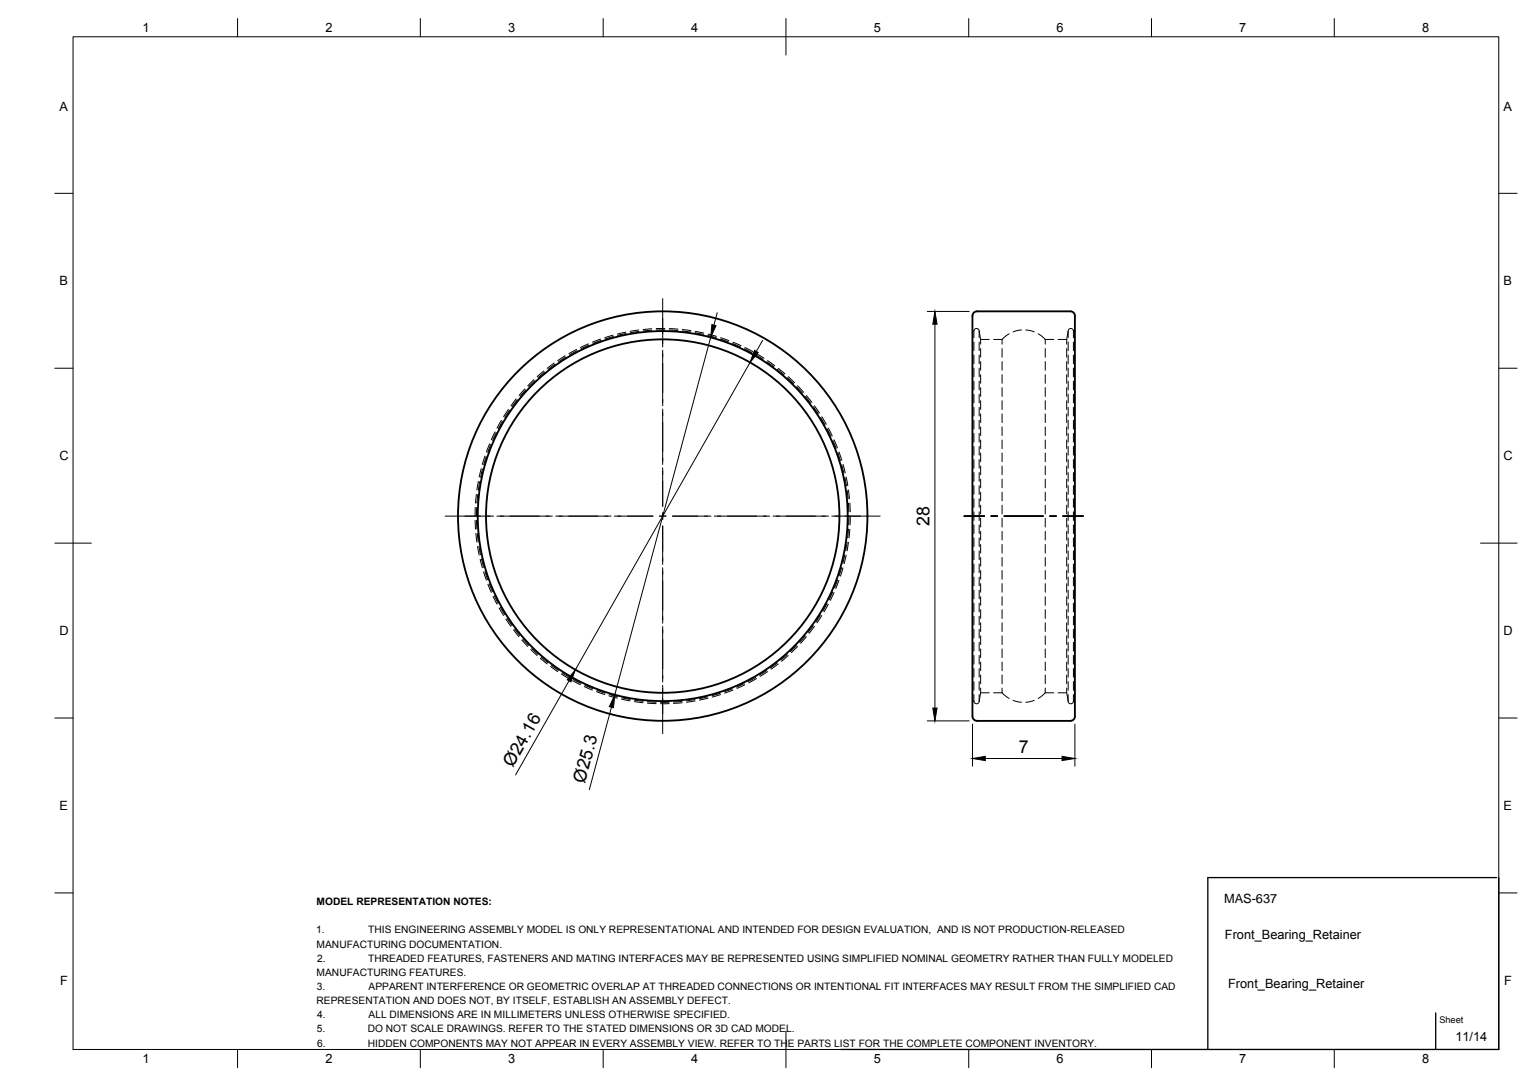
ISO-10303-21;
HEADER;
FILE_DESCRIPTION((''),'2;1');
FILE_NAME('Front_Bearing_Retainer.step','2026-10-09T10:11:57-07:00',(''),(''),'','','');
FILE_SCHEMA (('AUTOMOTIVE_DESIGN { 1 0 10303 214 3 1 1 }'));
ENDSEC;
DATA;
#10=MECHANICAL_DESIGN_GEOMETRIC_PRESENTATION_REPRESENTATION('',(#143),#13510);
#104=SHAPE_REPRESENTATION_RELATIONSHIP('SRR','None',#13574,#119) ;
#119=ADVANCED_BREP_SHAPE_REPRESENTATION('',(#175),#13506) ;
#143=STYLED_ITEM('',(#13650),#175) ;
#175=MANIFOLD_SOLID_BREP('Body1',#7392) ;
#254=FACE_BOUND('',#1570,.T.) ;
#255=FACE_BOUND('',#1572,.T.) ;
#462=PLANE('',#8395) ;
#463=PLANE('',#8396) ;
#516=TOROIDAL_SURFACE('',#8373,12.65,0.18) ;
#517=TOROIDAL_SURFACE('',#8378,13.7,0.3) ;
#518=TOROIDAL_SURFACE('',#8384,13.7,0.3) ;
#519=TOROIDAL_SURFACE('',#8390,12.65,0.18) ;
#520=TOROIDAL_SURFACE('',#8401,10.75,1.985) ;
#651=CYLINDRICAL_SURFACE('',#8376,12.65) ;
#652=CYLINDRICAL_SURFACE('',#8382,14.) ;
#653=CYLINDRICAL_SURFACE('',#8387,12.65) ;
#654=CYLINDRICAL_SURFACE('',#8397,12.08) ;
#655=CYLINDRICAL_SURFACE('',#8399,12.08) ;
#1045=FACE_OUTER_BOUND('',#1560,.T.) ;
#1046=FACE_OUTER_BOUND('',#1561,.T.) ;
#1047=FACE_OUTER_BOUND('',#1562,.T.) ;
#1048=FACE_OUTER_BOUND('',#1563,.T.) ;
#1049=FACE_OUTER_BOUND('',#1564,.T.) ;
#1050=FACE_OUTER_BOUND('',#1565,.T.) ;
#1051=FACE_OUTER_BOUND('',#1566,.T.) ;
#1052=FACE_OUTER_BOUND('',#1567,.T.) ;
#1053=FACE_OUTER_BOUND('',#1568,.T.) ;
#1054=FACE_OUTER_BOUND('',#1569,.T.) ;
#1055=FACE_OUTER_BOUND('',#1571,.T.) ;
#1056=FACE_OUTER_BOUND('',#1573,.T.) ;
#1057=FACE_OUTER_BOUND('',#1574,.T.) ;
#1058=FACE_OUTER_BOUND('',#1575,.T.) ;
#1560=EDGE_LOOP('',(#6604,#6605,#6606,#6607)) ;
#1561=EDGE_LOOP('',(#6608,#6609,#6610,#6611)) ;
#1562=EDGE_LOOP('',(#6612,#6613,#6614,#6615)) ;
#1563=EDGE_LOOP('',(#6616,#6617,#6618,#6619)) ;
#1564=EDGE_LOOP('',(#6620,#6621,#6622,#6623)) ;
#1565=EDGE_LOOP('',(#6624,#6625,#6626,#6627)) ;
#1566=EDGE_LOOP('',(#6628,#6629,#6630,#6631)) ;
#1567=EDGE_LOOP('',(#6632,#6633,#6634,#6635)) ;
#1568=EDGE_LOOP('',(#6636,#6637,#6638,#6639)) ;
#1569=EDGE_LOOP('',(#6640)) ;
#1570=EDGE_LOOP('',(#6641)) ;
#1571=EDGE_LOOP('',(#6642)) ;
#1572=EDGE_LOOP('',(#6643)) ;
#1573=EDGE_LOOP('',(#6644,#6645,#6646,#6647)) ;
#1574=EDGE_LOOP('',(#6648,#6649,#6650,#6651)) ;
#1575=EDGE_LOOP('',(#6652,#6653,#6654,#6655)) ;
#2112=LINE('',#13167,#2606) ;
#2113=LINE('',#13176,#2607) ;
#2114=LINE('',#13186,#2608) ;
#2115=LINE('',#13195,#2609) ;
#2116=LINE('',#13204,#2610) ;
#2117=LINE('',#13210,#2611) ;
#2118=LINE('',#13213,#2612) ;
#2606=VECTOR('',#10634,12.08) ;
#2607=VECTOR('',#10647,12.65) ;
#2608=VECTOR('',#10660,14.) ;
#2609=VECTOR('',#10671,12.65) ;
#2610=VECTOR('',#10684,12.08) ;
#2611=VECTOR('',#10693,12.08) ;
#2612=VECTOR('',#10696,12.08) ;
#3041=CIRCLE('',#8371,12.08) ;
#3042=CIRCLE('',#8372,12.65) ;
#3043=CIRCLE('',#8374,12.65) ;
#3044=CIRCLE('',#8375,0.18) ;
#3045=CIRCLE('',#8377,12.65) ;
#3046=CIRCLE('',#8379,14.) ;
#3047=CIRCLE('',#8380,0.3) ;
#3048=CIRCLE('',#8381,13.7) ;
#3049=CIRCLE('',#8383,14.) ;
#3050=CIRCLE('',#8385,13.7) ;
#3051=CIRCLE('',#8386,0.3) ;
#3052=CIRCLE('',#8388,12.65) ;
#3053=CIRCLE('',#8389,12.65) ;
#3054=CIRCLE('',#8391,12.65) ;
#3055=CIRCLE('',#8392,0.18) ;
#3056=CIRCLE('',#8394,12.08) ;
#3057=CIRCLE('',#8398,12.08) ;
#3058=CIRCLE('',#8400,12.08) ;
#3059=CIRCLE('',#8402,1.985) ;
#3712=VERTEX_POINT('',#13164) ;
#3713=VERTEX_POINT('',#13166) ;
#3714=VERTEX_POINT('',#13170) ;
#3715=VERTEX_POINT('',#13174) ;
#3716=VERTEX_POINT('',#13178) ;
#3717=VERTEX_POINT('',#13180) ;
#3718=VERTEX_POINT('',#13184) ;
#3719=VERTEX_POINT('',#13188) ;
#3720=VERTEX_POINT('',#13192) ;
#3721=VERTEX_POINT('',#13194) ;
#3722=VERTEX_POINT('',#13198) ;
#3723=VERTEX_POINT('',#13202) ;
#3724=VERTEX_POINT('',#13208) ;
#3725=VERTEX_POINT('',#13212) ;
#4689=EDGE_CURVE('',#3712,#3712,#3041,.F.) ;
#4690=EDGE_CURVE('',#3712,#3713,#2112,.T.) ;
#4691=EDGE_CURVE('',#3713,#3713,#3042,.F.) ;
#4692=EDGE_CURVE('',#3714,#3714,#3043,.T.) ;
#4693=EDGE_CURVE('',#3714,#3713,#3044,.T.) ;
#4694=EDGE_CURVE('',#3715,#3715,#3045,.T.) ;
#4695=EDGE_CURVE('',#3715,#3714,#2113,.T.) ;
#4696=EDGE_CURVE('',#3716,#3716,#3046,.T.) ;
#4697=EDGE_CURVE('',#3716,#3717,#3047,.T.) ;
#4698=EDGE_CURVE('',#3717,#3717,#3048,.T.) ;
#4699=EDGE_CURVE('',#3718,#3718,#3049,.T.) ;
#4700=EDGE_CURVE('',#3718,#3716,#2114,.T.) ;
#4701=EDGE_CURVE('',#3719,#3719,#3050,.T.) ;
#4702=EDGE_CURVE('',#3719,#3718,#3051,.T.) ;
#4703=EDGE_CURVE('',#3720,#3720,#3052,.T.) ;
#4704=EDGE_CURVE('',#3720,#3721,#2115,.T.) ;
#4705=EDGE_CURVE('',#3721,#3721,#3053,.T.) ;
#4706=EDGE_CURVE('',#3722,#3722,#3054,.T.) ;
#4707=EDGE_CURVE('',#3722,#3720,#3055,.T.) ;
#4708=EDGE_CURVE('',#3723,#3723,#3056,.T.) ;
#4709=EDGE_CURVE('',#3723,#3722,#2116,.T.) ;
#4710=EDGE_CURVE('',#3724,#3724,#3057,.T.) ;
#4711=EDGE_CURVE('',#3724,#3723,#2117,.T.) ;
#4712=EDGE_CURVE('',#3712,#3725,#2118,.T.) ;
#4713=EDGE_CURVE('',#3725,#3725,#3058,.T.) ;
#4714=EDGE_CURVE('',#3725,#3724,#3059,.T.) ;
#6604=ORIENTED_EDGE('',*,*,#4689,.T.) ;
#6605=ORIENTED_EDGE('',*,*,#4690,.T.) ;
#6606=ORIENTED_EDGE('',*,*,#4691,.F.) ;
#6607=ORIENTED_EDGE('',*,*,#4690,.F.) ;
#6608=ORIENTED_EDGE('',*,*,#4692,.F.) ;
#6609=ORIENTED_EDGE('',*,*,#4693,.T.) ;
#6610=ORIENTED_EDGE('',*,*,#4691,.T.) ;
#6611=ORIENTED_EDGE('',*,*,#4693,.F.) ;
#6612=ORIENTED_EDGE('',*,*,#4694,.F.) ;
#6613=ORIENTED_EDGE('',*,*,#4695,.T.) ;
#6614=ORIENTED_EDGE('',*,*,#4692,.T.) ;
#6615=ORIENTED_EDGE('',*,*,#4695,.F.) ;
#6616=ORIENTED_EDGE('',*,*,#4696,.F.) ;
#6617=ORIENTED_EDGE('',*,*,#4697,.T.) ;
#6618=ORIENTED_EDGE('',*,*,#4698,.T.) ;
#6619=ORIENTED_EDGE('',*,*,#4697,.F.) ;
#6620=ORIENTED_EDGE('',*,*,#4699,.F.) ;
#6621=ORIENTED_EDGE('',*,*,#4700,.T.) ;
#6622=ORIENTED_EDGE('',*,*,#4696,.T.) ;
#6623=ORIENTED_EDGE('',*,*,#4700,.F.) ;
#6624=ORIENTED_EDGE('',*,*,#4701,.F.) ;
#6625=ORIENTED_EDGE('',*,*,#4702,.T.) ;
#6626=ORIENTED_EDGE('',*,*,#4699,.T.) ;
#6627=ORIENTED_EDGE('',*,*,#4702,.F.) ;
#6628=ORIENTED_EDGE('',*,*,#4703,.F.) ;
#6629=ORIENTED_EDGE('',*,*,#4704,.T.) ;
#6630=ORIENTED_EDGE('',*,*,#4705,.T.) ;
#6631=ORIENTED_EDGE('',*,*,#4704,.F.) ;
#6632=ORIENTED_EDGE('',*,*,#4706,.F.) ;
#6633=ORIENTED_EDGE('',*,*,#4707,.T.) ;
#6634=ORIENTED_EDGE('',*,*,#4703,.T.) ;
#6635=ORIENTED_EDGE('',*,*,#4707,.F.) ;
#6636=ORIENTED_EDGE('',*,*,#4708,.F.) ;
#6637=ORIENTED_EDGE('',*,*,#4709,.T.) ;
#6638=ORIENTED_EDGE('',*,*,#4706,.T.) ;
#6639=ORIENTED_EDGE('',*,*,#4709,.F.) ;
#6640=ORIENTED_EDGE('',*,*,#4698,.F.) ;
#6641=ORIENTED_EDGE('',*,*,#4694,.T.) ;
#6642=ORIENTED_EDGE('',*,*,#4701,.T.) ;
#6643=ORIENTED_EDGE('',*,*,#4705,.F.) ;
#6644=ORIENTED_EDGE('',*,*,#4710,.F.) ;
#6645=ORIENTED_EDGE('',*,*,#4711,.T.) ;
#6646=ORIENTED_EDGE('',*,*,#4708,.T.) ;
#6647=ORIENTED_EDGE('',*,*,#4711,.F.) ;
#6648=ORIENTED_EDGE('',*,*,#4689,.F.) ;
#6649=ORIENTED_EDGE('',*,*,#4712,.T.) ;
#6650=ORIENTED_EDGE('',*,*,#4713,.T.) ;
#6651=ORIENTED_EDGE('',*,*,#4712,.F.) ;
#6652=ORIENTED_EDGE('',*,*,#4713,.F.) ;
#6653=ORIENTED_EDGE('',*,*,#4714,.T.) ;
#6654=ORIENTED_EDGE('',*,*,#4710,.T.) ;
#6655=ORIENTED_EDGE('',*,*,#4714,.F.) ;
#6904=CONICAL_SURFACE('',#8370,12.08,1.3962634016) ;
#6905=CONICAL_SURFACE('',#8393,12.08,1.3962634016) ;
#7295=ADVANCED_FACE('',(#1045),#6904,.F.) ;
#7296=ADVANCED_FACE('',(#1046),#516,.F.) ;
#7297=ADVANCED_FACE('',(#1047),#651,.F.) ;
#7298=ADVANCED_FACE('',(#1048),#517,.T.) ;
#7299=ADVANCED_FACE('',(#1049),#652,.T.) ;
#7300=ADVANCED_FACE('',(#1050),#518,.T.) ;
#7301=ADVANCED_FACE('',(#1051),#653,.F.) ;
#7302=ADVANCED_FACE('',(#1052),#519,.F.) ;
#7303=ADVANCED_FACE('',(#1053),#6905,.F.) ;
#7304=ADVANCED_FACE('',(#1054,#254),#462,.F.) ;
#7305=ADVANCED_FACE('',(#1055,#255),#463,.T.) ;
#7306=ADVANCED_FACE('',(#1056),#654,.F.) ;
#7307=ADVANCED_FACE('',(#1057),#655,.F.) ;
#7308=ADVANCED_FACE('',(#1058),#520,.F.) ;
#7392=CLOSED_SHELL('',(#7295,#7296,#7297,#7298,#7299,#7300,#7301,#7302,
#7303,#7304,#7305,#7306,#7307,#7308)) ;
#8369=AXIS2_PLACEMENT_3D('',#13162,#10628,#10629) ;
#8370=AXIS2_PLACEMENT_3D('',#13163,#10630,#10631) ;
#8371=AXIS2_PLACEMENT_3D('',#13165,#10632,#10633) ;
#8372=AXIS2_PLACEMENT_3D('',#13168,#10635,#10636) ;
#8373=AXIS2_PLACEMENT_3D('',#13169,#10637,#10638) ;
#8374=AXIS2_PLACEMENT_3D('',#13171,#10639,#10640) ;
#8375=AXIS2_PLACEMENT_3D('',#13172,#10641,#10642) ;
#8376=AXIS2_PLACEMENT_3D('',#13173,#10643,#10644) ;
#8377=AXIS2_PLACEMENT_3D('',#13175,#10645,#10646) ;
#8378=AXIS2_PLACEMENT_3D('',#13177,#10648,#10649) ;
#8379=AXIS2_PLACEMENT_3D('',#13179,#10650,#10651) ;
#8380=AXIS2_PLACEMENT_3D('',#13181,#10652,#10653) ;
#8381=AXIS2_PLACEMENT_3D('',#13182,#10654,#10655) ;
#8382=AXIS2_PLACEMENT_3D('',#13183,#10656,#10657) ;
#8383=AXIS2_PLACEMENT_3D('',#13185,#10658,#10659) ;
#8384=AXIS2_PLACEMENT_3D('',#13187,#10661,#10662) ;
#8385=AXIS2_PLACEMENT_3D('',#13189,#10663,#10664) ;
#8386=AXIS2_PLACEMENT_3D('',#13190,#10665,#10666) ;
#8387=AXIS2_PLACEMENT_3D('',#13191,#10667,#10668) ;
#8388=AXIS2_PLACEMENT_3D('',#13193,#10669,#10670) ;
#8389=AXIS2_PLACEMENT_3D('',#13196,#10672,#10673) ;
#8390=AXIS2_PLACEMENT_3D('',#13197,#10674,#10675) ;
#8391=AXIS2_PLACEMENT_3D('',#13199,#10676,#10677) ;
#8392=AXIS2_PLACEMENT_3D('',#13200,#10678,#10679) ;
#8393=AXIS2_PLACEMENT_3D('',#13201,#10680,#10681) ;
#8394=AXIS2_PLACEMENT_3D('',#13203,#10682,#10683) ;
#8395=AXIS2_PLACEMENT_3D('',#13205,#10685,#10686) ;
#8396=AXIS2_PLACEMENT_3D('',#13206,#10687,#10688) ;
#8397=AXIS2_PLACEMENT_3D('',#13207,#10689,#10690) ;
#8398=AXIS2_PLACEMENT_3D('',#13209,#10691,#10692) ;
#8399=AXIS2_PLACEMENT_3D('',#13211,#10694,#10695) ;
#8400=AXIS2_PLACEMENT_3D('',#13214,#10697,#10698) ;
#8401=AXIS2_PLACEMENT_3D('',#13215,#10699,#10700) ;
#8402=AXIS2_PLACEMENT_3D('',#13216,#10701,#10702) ;
#10628=DIRECTION('axis',(0.,0.,1.)) ;
#10629=DIRECTION('refdir',(1.,0.,0.)) ;
#10630=DIRECTION('center_axis',(0.,0.,1.)) ;
#10631=DIRECTION('ref_axis',(0.877582561890372,-0.479425538604204,0.)) ;
#10632=DIRECTION('center_axis',(0.,0.,1.)) ;
#10633=DIRECTION('ref_axis',(-1.,0.,0.)) ;
#10634=DIRECTION('',(-0.864250110858646,0.472141987409851,0.173648177662463)) ;
#10635=DIRECTION('center_axis',(0.,0.,1.)) ;
#10636=DIRECTION('ref_axis',(-1.,0.,0.)) ;
#10637=DIRECTION('center_axis',(0.,0.,-1.)) ;
#10638=DIRECTION('ref_axis',(0.877582561890372,-0.479425538604204,0.)) ;
#10639=DIRECTION('center_axis',(0.,0.,-1.)) ;
#10640=DIRECTION('ref_axis',(1.,0.,0.)) ;
#10641=DIRECTION('center_axis',(-0.479425538604204,-0.877582561890372,0.)) ;
#10642=DIRECTION('ref_axis',(-0.877582561890372,0.479425538604204,0.)) ;
#10643=DIRECTION('center_axis',(0.,0.,-1.)) ;
#10644=DIRECTION('ref_axis',(0.877582561890372,-0.479425538604204,0.)) ;
#10645=DIRECTION('center_axis',(0.,0.,-1.)) ;
#10646=DIRECTION('ref_axis',(1.,0.,0.)) ;
#10647=DIRECTION('',(0.,0.,-1.)) ;
#10648=DIRECTION('center_axis',(0.,0.,-1.)) ;
#10649=DIRECTION('ref_axis',(0.877582561890372,-0.479425538604204,0.)) ;
#10650=DIRECTION('center_axis',(0.,0.,-1.)) ;
#10651=DIRECTION('ref_axis',(1.,0.,0.)) ;
#10652=DIRECTION('center_axis',(0.479425538604204,0.877582561890372,0.)) ;
#10653=DIRECTION('ref_axis',(-0.877582561890372,0.479425538604204,0.)) ;
#10654=DIRECTION('center_axis',(0.,0.,-1.)) ;
#10655=DIRECTION('ref_axis',(1.,0.,0.)) ;
#10656=DIRECTION('center_axis',(0.,0.,-1.)) ;
#10657=DIRECTION('ref_axis',(0.877582561890372,-0.479425538604204,0.)) ;
#10658=DIRECTION('center_axis',(0.,0.,-1.)) ;
#10659=DIRECTION('ref_axis',(1.,0.,0.)) ;
#10660=DIRECTION('',(0.,0.,1.)) ;
#10661=DIRECTION('center_axis',(0.,0.,-1.)) ;
#10662=DIRECTION('ref_axis',(0.877582561890372,-0.479425538604204,0.)) ;
#10663=DIRECTION('center_axis',(0.,0.,-1.)) ;
#10664=DIRECTION('ref_axis',(1.,0.,0.)) ;
#10665=DIRECTION('center_axis',(0.479425538604204,0.877582561890372,0.)) ;
#10666=DIRECTION('ref_axis',(-0.877582561890372,0.479425538604204,0.)) ;
#10667=DIRECTION('center_axis',(0.,0.,-1.)) ;
#10668=DIRECTION('ref_axis',(0.877582561890372,-0.479425538604204,0.)) ;
#10669=DIRECTION('center_axis',(0.,0.,-1.)) ;
#10670=DIRECTION('ref_axis',(1.,0.,0.)) ;
#10671=DIRECTION('',(0.,0.,-1.)) ;
#10672=DIRECTION('center_axis',(0.,0.,-1.)) ;
#10673=DIRECTION('ref_axis',(1.,0.,0.)) ;
#10674=DIRECTION('center_axis',(0.,0.,-1.)) ;
#10675=DIRECTION('ref_axis',(0.877582561890372,-0.479425538604204,0.)) ;
#10676=DIRECTION('center_axis',(0.,0.,-1.)) ;
#10677=DIRECTION('ref_axis',(1.,0.,0.)) ;
#10678=DIRECTION('center_axis',(-0.479425538604204,-0.877582561890372,0.)) ;
#10679=DIRECTION('ref_axis',(-0.877582561890372,0.479425538604204,0.)) ;
#10680=DIRECTION('center_axis',(0.,0.,-1.)) ;
#10681=DIRECTION('ref_axis',(0.877582561890372,-0.479425538604204,0.)) ;
#10682=DIRECTION('center_axis',(0.,0.,-1.)) ;
#10683=DIRECTION('ref_axis',(1.,0.,0.)) ;
#10684=DIRECTION('',(-0.864250110858646,0.472141987409851,-0.173648177662463)) ;
#10685=DIRECTION('center_axis',(0.,0.,-1.)) ;
#10686=DIRECTION('ref_axis',(1.,0.,0.)) ;
#10687=DIRECTION('center_axis',(0.,0.,-1.)) ;
#10688=DIRECTION('ref_axis',(1.,0.,0.)) ;
#10689=DIRECTION('center_axis',(0.,0.,-1.)) ;
#10690=DIRECTION('ref_axis',(0.877582561890372,-0.479425538604204,0.)) ;
#10691=DIRECTION('center_axis',(0.,0.,-1.)) ;
#10692=DIRECTION('ref_axis',(1.,0.,0.)) ;
#10693=DIRECTION('',(0.,0.,-1.)) ;
#10694=DIRECTION('center_axis',(0.,0.,-1.)) ;
#10695=DIRECTION('ref_axis',(0.877582561890372,-0.479425538604204,0.)) ;
#10696=DIRECTION('',(0.,0.,-1.)) ;
#10697=DIRECTION('center_axis',(0.,0.,-1.)) ;
#10698=DIRECTION('ref_axis',(1.,0.,0.)) ;
#10699=DIRECTION('center_axis',(0.,0.,-1.)) ;
#10700=DIRECTION('ref_axis',(0.877582561890372,-0.479425538604204,0.)) ;
#10701=DIRECTION('center_axis',(-0.479425538604204,-0.877582561890372,0.)) ;
#10702=DIRECTION('ref_axis',(-0.877582561890372,0.479425538604204,0.)) ;
#13162=CARTESIAN_POINT('',(0.,0.,0.)) ;
#13163=CARTESIAN_POINT('Origin',(0.,0.,9.439493621)) ;
#13164=CARTESIAN_POINT('',(-10.6011973476357,5.79146050633878,9.439493621)) ;
#13165=CARTESIAN_POINT('Origin',(0.,0.,9.439493621)) ;
#13166=CARTESIAN_POINT('',(-11.101419407913,6.06473306334308,9.54000000000113)) ;
#13167=CARTESIAN_POINT('',(-10.6011973476357,5.79146050633878,9.439493621)) ;
#13168=CARTESIAN_POINT('Origin',(0.,0.,9.54)) ;
#13169=CARTESIAN_POINT('Origin',(0.,0.,9.72)) ;
#13170=CARTESIAN_POINT('',(-11.1014194079132,6.06473306334318,9.9)) ;
#13171=CARTESIAN_POINT('Origin',(0.,0.,9.9)) ;
#13172=CARTESIAN_POINT('Origin',(-11.1014194079132,6.06473306334318,9.72)) ;
#13173=CARTESIAN_POINT('Origin',(0.,0.,6.50000000002)) ;
#13174=CARTESIAN_POINT('',(-11.1014194079132,6.06473306334318,10.)) ;
#13175=CARTESIAN_POINT('Origin',(0.,0.,10.)) ;
#13176=CARTESIAN_POINT('',(-11.1014194079132,6.06473306334318,6.50000000002)) ;
#13177=CARTESIAN_POINT('Origin',(0.,0.,9.7)) ;
#13178=CARTESIAN_POINT('',(-12.2861558664652,6.71195754045885,9.7)) ;
#13179=CARTESIAN_POINT('Origin',(0.,0.,9.7)) ;
#13180=CARTESIAN_POINT('',(-12.0228810978981,6.56812987887759,10.)) ;
#13181=CARTESIAN_POINT('Origin',(-12.0228810978981,6.5681298788776,9.7)) ;
#13182=CARTESIAN_POINT('Origin',(0.,0.,10.)) ;
#13183=CARTESIAN_POINT('Origin',(0.,0.,6.50000000002)) ;
#13184=CARTESIAN_POINT('',(-12.2861558664652,6.71195754045885,3.3)) ;
#13185=CARTESIAN_POINT('Origin',(0.,0.,3.3)) ;
#13186=CARTESIAN_POINT('',(-12.2861558664652,6.71195754045886,6.50000000002)) ;
#13187=CARTESIAN_POINT('Origin',(0.,0.,3.3)) ;
#13188=CARTESIAN_POINT('',(-12.0228810978981,6.56812987887759,3.)) ;
#13189=CARTESIAN_POINT('Origin',(0.,0.,3.)) ;
#13190=CARTESIAN_POINT('Origin',(-12.0228810978981,6.5681298788776,3.3)) ;
#13191=CARTESIAN_POINT('Origin',(0.,0.,6.50000000002)) ;
#13192=CARTESIAN_POINT('',(-11.1014194079132,6.06473306334318,3.1)) ;
#13193=CARTESIAN_POINT('Origin',(0.,0.,3.1)) ;
#13194=CARTESIAN_POINT('',(-11.1014194079132,6.06473306334318,3.)) ;
#13195=CARTESIAN_POINT('',(-11.1014194079132,6.06473306334318,6.50000000002)) ;
#13196=CARTESIAN_POINT('Origin',(0.,0.,3.)) ;
#13197=CARTESIAN_POINT('Origin',(0.,0.,3.28)) ;
#13198=CARTESIAN_POINT('',(-11.1014194079132,6.06473306334318,3.46)) ;
#13199=CARTESIAN_POINT('Origin',(0.,0.,3.46)) ;
#13200=CARTESIAN_POINT('Origin',(-11.1014194079132,6.06473306334318,3.28)) ;
#13201=CARTESIAN_POINT('Origin',(0.,0.,3.560506379)) ;
#13202=CARTESIAN_POINT('',(-10.6011973476357,5.79146050633878,3.560506379)) ;
#13203=CARTESIAN_POINT('Origin',(0.,0.,3.560506379)) ;
#13204=CARTESIAN_POINT('',(-10.6011973476357,5.79146050633879,3.560506379)) ;
#13205=CARTESIAN_POINT('Origin',(7.8,0.,10.)) ;
#13206=CARTESIAN_POINT('Origin',(7.8,0.,3.)) ;
#13207=CARTESIAN_POINT('Origin',(0.,0.,6.50000000002)) ;
#13208=CARTESIAN_POINT('',(-10.6011973476,5.79146050634,5.02645834806)) ;
#13209=CARTESIAN_POINT('Origin',(0.,0.,5.02645834806)) ;
#13210=CARTESIAN_POINT('',(-10.6011973476357,5.79146050633879,6.50000000002)) ;
#13211=CARTESIAN_POINT('Origin',(0.,0.,6.50000000002)) ;
#13212=CARTESIAN_POINT('',(-10.6011973476,5.79146050634,7.97354165194)) ;
#13213=CARTESIAN_POINT('',(-10.6011973476357,5.79146050633879,6.50000000002)) ;
#13214=CARTESIAN_POINT('Origin',(0.,0.,7.97354165194)) ;
#13215=CARTESIAN_POINT('Origin',(0.,0.,6.5)) ;
#13216=CARTESIAN_POINT('Origin',(-9.4340125403215,5.15382453999519,6.5)) ;
#13489=UNCERTAINTY_MEASURE_WITH_UNIT(LENGTH_MEASURE(0.01),#13511,
'DISTANCE_ACCURACY_VALUE',
'Maximum model space distance between geometric entities at asserted c
onnectivities') ;
#13493=UNCERTAINTY_MEASURE_WITH_UNIT(LENGTH_MEASURE(0.01),#13511,
'DISTANCE_ACCURACY_VALUE',
'Maximum model space distance between geometric entities at asserted c
onnectivities') ;
#13506=(
GEOMETRIC_REPRESENTATION_CONTEXT(3)
GLOBAL_UNCERTAINTY_ASSIGNED_CONTEXT((#13489))
GLOBAL_UNIT_ASSIGNED_CONTEXT((#13511,#13513,#13514))
REPRESENTATION_CONTEXT('','3D')
) ;
#13510=(
GEOMETRIC_REPRESENTATION_CONTEXT(3)
GLOBAL_UNCERTAINTY_ASSIGNED_CONTEXT((#13493))
GLOBAL_UNIT_ASSIGNED_CONTEXT((#13511,#13513,#13514))
REPRESENTATION_CONTEXT('','3D')
) ;
#13511=(
LENGTH_UNIT()
NAMED_UNIT(*)
SI_UNIT(.MILLI.,.METRE.)
) ;
#13513=(
NAMED_UNIT(*)
PLANE_ANGLE_UNIT()
SI_UNIT($,.RADIAN.)
) ;
#13514=(
NAMED_UNIT(*)
SI_UNIT($,.STERADIAN.)
SOLID_ANGLE_UNIT()
) ;
#13527=SHAPE_DEFINITION_REPRESENTATION(#13543,#13574) ;
#13543=PRODUCT_DEFINITION_SHAPE('',$,#13591) ;
#13574=SHAPE_REPRESENTATION('',(#8369),#13506) ;
#13578=PRODUCT_DEFINITION_CONTEXT('part definition',#13628,'design') ;
#13591=PRODUCT_DEFINITION('Front_Bearing_Retainer',
'Front_Bearing_Retainer',#13607,#13578) ;
#13607=PRODUCT_DEFINITION_FORMATION('',$,#13642) ;
#13628=APPLICATION_CONTEXT(
'Core Data for Automotive Mechanical Design Process') ;
#13629=PRODUCT_CONTEXT('part definition',#13628,'mechanical') ;
#13642=PRODUCT('Front_Bearing_Retainer','Front_Bearing_Retainer',$,(#13629)) ;
#13650=PRESENTATION_STYLE_ASSIGNMENT((#13655)) ;
#13655=SURFACE_STYLE_USAGE(.BOTH.,#13660) ;
#13660=SURFACE_SIDE_STYLE('',(#13665)) ;
#13665=SURFACE_STYLE_FILL_AREA(#13670) ;
#13670=FILL_AREA_STYLE('Opaque(144,144,144)',(#13675)) ;
#13675=FILL_AREA_STYLE_COLOUR('Opaque(144,144,144)',#13680) ;
#13680=COLOUR_RGB('Opaque(144,144,144)', 0.40784314, 0.44705882, 0.49803922) ;
ENDSEC;
END-ISO-10303-21;
